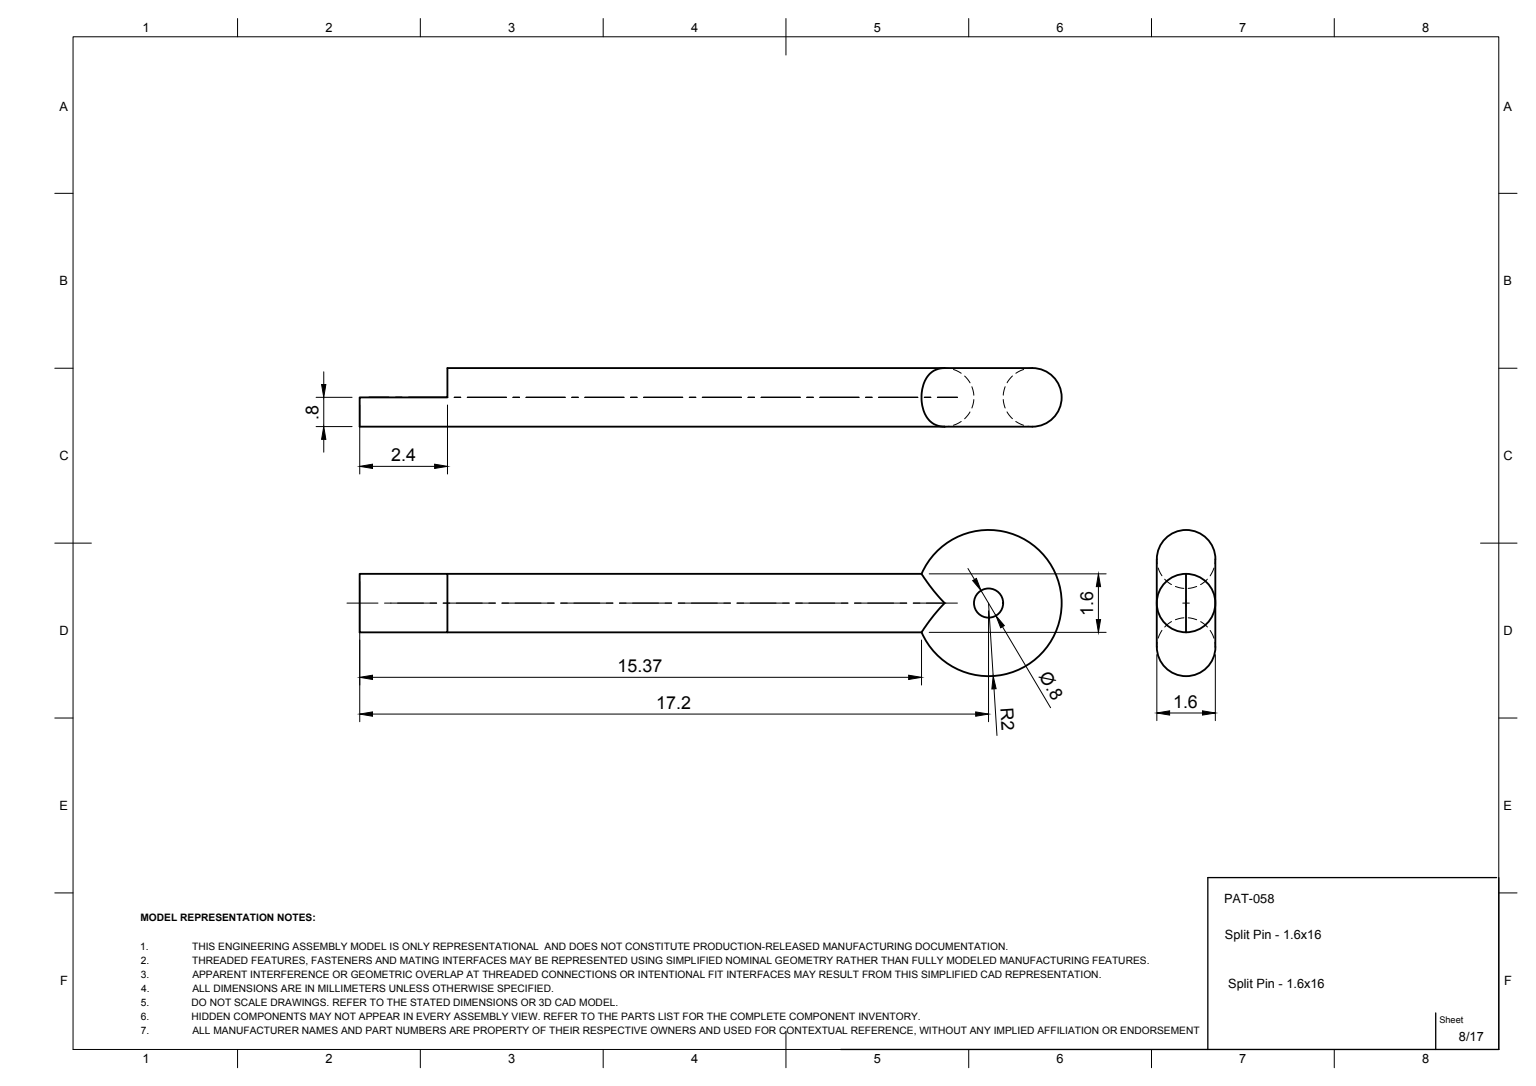
ISO-10303-21;
HEADER;
/* Generated by software containing ST-Developer
 * from STEP Tools, Inc. (www.steptools.com) 
 */

FILE_DESCRIPTION(
/* description */ ('Horizontal push-pull toggle clamp'),
/* implementation_level */ '2;1');

FILE_NAME(
/* name */ 'Split Pin - 1.6x16.step',
/* time_stamp */ '2026-10-27T21:21:09-07:00',
/* author */ (''),
/* organization */ (''),
/* preprocessor_version */ 'ST-DEVELOPER v20.2',
/* originating_system */ 'Autodesk Translation Framework v15.17.0.0',
/* authorisation */ '');

FILE_SCHEMA (('AUTOMOTIVE_DESIGN { 1 0 10303 214 3 1 1 }'));
ENDSEC;

DATA;
#10=MECHANICAL_DESIGN_GEOMETRIC_PRESENTATION_REPRESENTATION('',(#197),#4791);
#11=TOROIDAL_SURFACE('',#3033,0.12,0.08);
#16=B_SPLINE_CURVE_WITH_KNOTS('',3,(#4658,#4659,#4660,#4661,#4662,#4663,
#4664,#4665,#4666,#4667,#4668,#4669,#4670,#4671,#4672,#4673,#4674,#4675,
#4676,#4677,#4678,#4679,#4680,#4681,#4682,#4683),.UNSPECIFIED.,.F.,.F.,
(4,2,2,2,2,2,2,2,2,2,2,2,4),(-0.00054581412719389,0.,0.0281583564005144,
0.0618496465371181,0.0905865724114538,0.120694112793616,0.144966158459363,
0.16923820412511,0.199345744507272,0.228082670381608,0.261773960518212,
0.289932316918681,0.290478131045882),.UNSPECIFIED.);
#17=B_SPLINE_CURVE_WITH_KNOTS('',3,(#4684,#4685,#4686,#4687,#4688,#4689,
#4690,#4691,#4692,#4693,#4694,#4695,#4696,#4697,#4698,#4699,#4700,#4701,
#4702,#4703,#4704,#4705,#4706,#4707,#4708,#4709),.UNSPECIFIED.,.F.,.F.,
(4,2,2,2,2,2,2,2,2,2,2,2,4),(-0.000545814127196571,0.,0.0281583564006391,
0.0618496465374156,0.0905865724118984,0.120694112794215,0.144966158460086,
0.169238204125958,0.199345744508275,0.228082670382758,0.261773960519534,
0.289932316920171,0.29047813104737),.UNSPECIFIED.);
#171=SHAPE_REPRESENTATION_RELATIONSHIP('SRR','None',#4877,#184);
#184=ADVANCED_BREP_SHAPE_REPRESENTATION('',(#209),#4790);
#197=STYLED_ITEM('',(#5023),#209);
#209=MANIFOLD_SOLID_BREP('Body1',#2642);
#255=FACE_BOUND('',#705,.T.);
#359=PLANE('',#3036);
#360=PLANE('',#3038);
#361=PLANE('',#3042);
#508=FACE_OUTER_BOUND('',#704,.T.);
#509=FACE_OUTER_BOUND('',#706,.T.);
#510=FACE_OUTER_BOUND('',#707,.T.);
#511=FACE_OUTER_BOUND('',#708,.T.);
#512=FACE_OUTER_BOUND('',#709,.T.);
#704=EDGE_LOOP('',(#2419,#2420,#2421,#2422));
#705=EDGE_LOOP('',(#2423,#2424));
#706=EDGE_LOOP('',(#2425,#2426));
#707=EDGE_LOOP('',(#2427,#2428,#2429,#2430));
#708=EDGE_LOOP('',(#2431,#2432,#2433,#2434,#2435,#2436,#2437,#2438,#2439));
#709=EDGE_LOOP('',(#2440,#2441,#2442));
#791=CIRCLE('',#3034,0.08);
#792=CIRCLE('',#3035,0.04);
#793=CIRCLE('',#3037,0.08);
#794=CIRCLE('',#3040,0.08);
#795=CIRCLE('',#3041,0.08);
#1011=LINE('',#4714,#1231);
#1012=LINE('',#4717,#1232);
#1013=LINE('',#4719,#1233);
#1014=LINE('',#4720,#1234);
#1015=LINE('',#4724,#1235);
#1231=VECTOR('',#3787,1.);
#1232=VECTOR('',#3790,1.);
#1233=VECTOR('',#3791,1.);
#1234=VECTOR('',#3792,1.);
#1235=VECTOR('',#3797,0.08);
#1445=VERTEX_POINT('',#4653);
#1446=VERTEX_POINT('',#4656);
#1447=VERTEX_POINT('',#4657);
#1448=VERTEX_POINT('',#4711);
#1449=VERTEX_POINT('',#4712);
#1450=VERTEX_POINT('',#4716);
#1451=VERTEX_POINT('',#4718);
#1452=VERTEX_POINT('',#4722);
#1771=EDGE_CURVE('',#1445,#1445,#791,.T.);
#1772=EDGE_CURVE('',#1445,#1445,#792,.T.);
#1773=EDGE_CURVE('',#1446,#1447,#16,.T.);
#1774=EDGE_CURVE('',#1447,#1446,#17,.T.);
#1775=EDGE_CURVE('',#1448,#1449,#793,.T.);
#1776=EDGE_CURVE('',#1448,#1449,#1011,.T.);
#1777=EDGE_CURVE('',#1449,#1450,#1012,.T.);
#1778=EDGE_CURVE('',#1451,#1450,#1013,.T.);
#1779=EDGE_CURVE('',#1448,#1451,#1014,.T.);
#1780=EDGE_CURVE('',#1452,#1451,#794,.T.);
#1781=EDGE_CURVE('',#1452,#1447,#1015,.T.);
#1782=EDGE_CURVE('',#1450,#1452,#795,.T.);
#2419=ORIENTED_EDGE('',*,*,#1771,.F.);
#2420=ORIENTED_EDGE('',*,*,#1772,.T.);
#2421=ORIENTED_EDGE('',*,*,#1771,.T.);
#2422=ORIENTED_EDGE('',*,*,#1772,.F.);
#2423=ORIENTED_EDGE('',*,*,#1773,.F.);
#2424=ORIENTED_EDGE('',*,*,#1774,.F.);
#2425=ORIENTED_EDGE('',*,*,#1775,.T.);
#2426=ORIENTED_EDGE('',*,*,#1776,.F.);
#2427=ORIENTED_EDGE('',*,*,#1776,.T.);
#2428=ORIENTED_EDGE('',*,*,#1777,.T.);
#2429=ORIENTED_EDGE('',*,*,#1778,.F.);
#2430=ORIENTED_EDGE('',*,*,#1779,.F.);
#2431=ORIENTED_EDGE('',*,*,#1775,.F.);
#2432=ORIENTED_EDGE('',*,*,#1779,.T.);
#2433=ORIENTED_EDGE('',*,*,#1780,.F.);
#2434=ORIENTED_EDGE('',*,*,#1781,.T.);
#2435=ORIENTED_EDGE('',*,*,#1774,.T.);
#2436=ORIENTED_EDGE('',*,*,#1773,.T.);
#2437=ORIENTED_EDGE('',*,*,#1781,.F.);
#2438=ORIENTED_EDGE('',*,*,#1782,.F.);
#2439=ORIENTED_EDGE('',*,*,#1777,.F.);
#2440=ORIENTED_EDGE('',*,*,#1782,.T.);
#2441=ORIENTED_EDGE('',*,*,#1780,.T.);
#2442=ORIENTED_EDGE('',*,*,#1778,.T.);
#2477=CYLINDRICAL_SURFACE('',#3039,0.08);
#2624=ADVANCED_FACE('',(#508,#255),#11,.T.);
#2625=ADVANCED_FACE('',(#509),#359,.F.);
#2626=ADVANCED_FACE('',(#510),#360,.T.);
#2627=ADVANCED_FACE('',(#511),#2477,.T.);
#2628=ADVANCED_FACE('',(#512),#361,.F.);
#2642=CLOSED_SHELL('',(#2624,#2625,#2626,#2627,#2628));
#3032=AXIS2_PLACEMENT_3D('',#4651,#3775,#3776);
#3033=AXIS2_PLACEMENT_3D('',#4652,#3777,#3778);
#3034=AXIS2_PLACEMENT_3D('',#4654,#3779,#3780);
#3035=AXIS2_PLACEMENT_3D('',#4655,#3781,#3782);
#3036=AXIS2_PLACEMENT_3D('',#4710,#3783,#3784);
#3037=AXIS2_PLACEMENT_3D('',#4713,#3785,#3786);
#3038=AXIS2_PLACEMENT_3D('',#4715,#3788,#3789);
#3039=AXIS2_PLACEMENT_3D('',#4721,#3793,#3794);
#3040=AXIS2_PLACEMENT_3D('',#4723,#3795,#3796);
#3041=AXIS2_PLACEMENT_3D('',#4725,#3798,#3799);
#3042=AXIS2_PLACEMENT_3D('',#4726,#3800,#3801);
#3775=DIRECTION('axis',(0.,0.,1.));
#3776=DIRECTION('refdir',(1.,0.,0.));
#3777=DIRECTION('center_axis',(-1.,0.,0.));
#3778=DIRECTION('ref_axis',(0.,0.,1.));
#3779=DIRECTION('center_axis',(0.,-1.,1.38777878078145E-16));
#3780=DIRECTION('ref_axis',(0.,-1.38777878078145E-16,-1.));
#3781=DIRECTION('center_axis',(1.,0.,0.));
#3782=DIRECTION('ref_axis',(0.,0.,1.));
#3783=DIRECTION('center_axis',(0.,1.,0.));
#3784=DIRECTION('ref_axis',(1.,0.,0.));
#3785=DIRECTION('center_axis',(0.,-1.,0.));
#3786=DIRECTION('ref_axis',(1.,0.,0.));
#3787=DIRECTION('',(0.,0.,1.));
#3788=DIRECTION('center_axis',(1.,0.,0.));
#3789=DIRECTION('ref_axis',(0.,0.,1.));
#3790=DIRECTION('',(0.,-1.,0.));
#3791=DIRECTION('',(0.,0.,1.));
#3792=DIRECTION('',(0.,-1.,0.));
#3793=DIRECTION('center_axis',(0.,-1.,0.));
#3794=DIRECTION('ref_axis',(1.,0.,0.));
#3795=DIRECTION('center_axis',(0.,-1.,0.));
#3796=DIRECTION('ref_axis',(1.,0.,0.));
#3797=DIRECTION('',(0.,1.,0.));
#3798=DIRECTION('center_axis',(0.,-1.,0.));
#3799=DIRECTION('ref_axis',(1.,0.,0.));
#3800=DIRECTION('center_axis',(0.,1.,0.));
#3801=DIRECTION('ref_axis',(1.,0.,0.));
#4651=CARTESIAN_POINT('',(0.,0.,0.));
#4652=CARTESIAN_POINT('Origin',(0.,0.12,0.));
#4653=CARTESIAN_POINT('',(-9.79717439317883E-18,0.12,-0.04));
#4654=CARTESIAN_POINT('Origin',(0.,0.12,-0.12));
#4655=CARTESIAN_POINT('Origin',(9.79717439317883E-18,0.12,0.));
#4656=CARTESIAN_POINT('',(0.08,-4.89858719658941E-18,7.34788079488412E-18));
#4657=CARTESIAN_POINT('',(-0.08,-4.89858719658941E-18,7.34788079488412E-18));
#4658=CARTESIAN_POINT('Ctrl Pts',(0.08,-4.89858719658941E-18,7.34788079488412E-18));
#4659=CARTESIAN_POINT('Ctrl Pts',(0.08,-0.00012864962353541,0.000128649623535413));
#4660=CARTESIAN_POINT('Ctrl Pts',(0.0799996896739287,-0.00025719571182076,
0.000257402596003253));
#4661=CARTESIAN_POINT('Ctrl Pts',(0.0799669711262291,-0.00701193164572964,
0.00703384588894362));
#4662=CARTESIAN_POINT('Ctrl Pts',(0.0791054994909294,-0.0133457972655825,
0.0139383126556792));
#4663=CARTESIAN_POINT('Ctrl Pts',(0.0749700088488058,-0.0265076530862524,
0.0292212026164895));
#4664=CARTESIAN_POINT('Ctrl Pts',(0.0712702072865517,-0.0331317062461458,
0.0375603420117568));
#4665=CARTESIAN_POINT('Ctrl Pts',(0.0612858949407667,-0.0440683985740427,
0.0520545604187517));
#4666=CARTESIAN_POINT('Ctrl Pts',(0.0555090276731744,-0.0485199197794574,
0.0582717815295611));
#4667=CARTESIAN_POINT('Ctrl Pts',(0.0412398082144208,-0.0561090538733877,
0.0691638397919718));
#4668=CARTESIAN_POINT('Ctrl Pts',(0.0327878980890048,-0.059089642483296,
0.0736229049587921));
#4669=CARTESIAN_POINT('Ctrl Pts',(0.0159233027310102,-0.0625179833270725,
0.0787936360751706));
#4670=CARTESIAN_POINT('Ctrl Pts',(0.00801661414593076,-0.0633030277982336,
0.08));
#4671=CARTESIAN_POINT('Ctrl Pts',(-0.00801661414593074,-0.0633030277982336,
0.08));
#4672=CARTESIAN_POINT('Ctrl Pts',(-0.0159233027310102,-0.0625179833270726,
0.0787936360751706));
#4673=CARTESIAN_POINT('Ctrl Pts',(-0.0327878980890049,-0.059089642483296,
0.0736229049587921));
#4674=CARTESIAN_POINT('Ctrl Pts',(-0.0412398082144209,-0.0561090538733877,
0.0691638397919717));
#4675=CARTESIAN_POINT('Ctrl Pts',(-0.0555090276731744,-0.0485199197794574,
0.0582717815295611));
#4676=CARTESIAN_POINT('Ctrl Pts',(-0.0612858949407667,-0.0440683985740427,
0.0520545604187517));
#4677=CARTESIAN_POINT('Ctrl Pts',(-0.0712702072865517,-0.0331317062461458,
0.0375603420117568));
#4678=CARTESIAN_POINT('Ctrl Pts',(-0.0749700088488058,-0.0265076530862524,
0.0292212026164895));
#4679=CARTESIAN_POINT('Ctrl Pts',(-0.0791054994909264,-0.0133457972655921,
0.0139383126556903));
#4680=CARTESIAN_POINT('Ctrl Pts',(-0.0799669711262287,-0.00701193164579759,
0.0070338458890125));
#4681=CARTESIAN_POINT('Ctrl Pts',(-0.0799996896739287,-0.000257195711817665,
0.000257402596000083));
#4682=CARTESIAN_POINT('Ctrl Pts',(-0.08,-0.000128649623538514,0.000128649623538516));
#4683=CARTESIAN_POINT('Ctrl Pts',(-0.08,-4.89858719658941E-18,7.34788079488412E-18));
#4684=CARTESIAN_POINT('Ctrl Pts',(-0.08,-4.89858719658941E-18,7.34788079488412E-18));
#4685=CARTESIAN_POINT('Ctrl Pts',(-0.08,-0.000128649623536042,-0.00012864962353603));
#4686=CARTESIAN_POINT('Ctrl Pts',(-0.0799996896739287,-0.000257195711820127,
-0.000257402596002604));
#4687=CARTESIAN_POINT('Ctrl Pts',(-0.0799669711262289,-0.0070119316457589,
-0.00703384588897312));
#4688=CARTESIAN_POINT('Ctrl Pts',(-0.0791054994909281,-0.0133457972655867,
-0.0139383126556841));
#4689=CARTESIAN_POINT('Ctrl Pts',(-0.0749700088488058,-0.0265076530862525,
-0.0292212026164896));
#4690=CARTESIAN_POINT('Ctrl Pts',(-0.0712702072865516,-0.0331317062461459,
-0.0375603420117568));
#4691=CARTESIAN_POINT('Ctrl Pts',(-0.0612858949407667,-0.0440683985740427,
-0.0520545604187517));
#4692=CARTESIAN_POINT('Ctrl Pts',(-0.0555090276731744,-0.0485199197794574,
-0.0582717815295611));
#4693=CARTESIAN_POINT('Ctrl Pts',(-0.0412398082144209,-0.0561090538733877,
-0.0691638397919717));
#4694=CARTESIAN_POINT('Ctrl Pts',(-0.0327878980890049,-0.059089642483296,
-0.0736229049587921));
#4695=CARTESIAN_POINT('Ctrl Pts',(-0.0159233027310101,-0.0625179833270725,
-0.0787936360751706));
#4696=CARTESIAN_POINT('Ctrl Pts',(-0.00801661414593069,-0.0633030277982336,
-0.08));
#4697=CARTESIAN_POINT('Ctrl Pts',(0.0080166141459307,-0.0633030277982336,
-0.08));
#4698=CARTESIAN_POINT('Ctrl Pts',(0.0159233027310101,-0.0625179833270725,
-0.0787936360751706));
#4699=CARTESIAN_POINT('Ctrl Pts',(0.0327878980890049,-0.0590896424832959,
-0.0736229049587921));
#4700=CARTESIAN_POINT('Ctrl Pts',(0.0412398082144209,-0.0561090538733877,
-0.0691638397919717));
#4701=CARTESIAN_POINT('Ctrl Pts',(0.0555090276731744,-0.0485199197794574,
-0.0582717815295611));
#4702=CARTESIAN_POINT('Ctrl Pts',(0.0612858949407666,-0.0440683985740428,
-0.0520545604187518));
#4703=CARTESIAN_POINT('Ctrl Pts',(0.0712702072865517,-0.0331317062461458,
-0.0375603420117568));
#4704=CARTESIAN_POINT('Ctrl Pts',(0.0749700088488058,-0.0265076530862524,
-0.0292212026164895));
#4705=CARTESIAN_POINT('Ctrl Pts',(0.079105499490928,-0.013345797265587,
-0.0139383126556845));
#4706=CARTESIAN_POINT('Ctrl Pts',(0.0799669711262289,-0.00701193164576148,
-0.00703384588897579));
#4707=CARTESIAN_POINT('Ctrl Pts',(0.0799996896739287,-0.000257195711819584,
-0.000257402596002039));
#4708=CARTESIAN_POINT('Ctrl Pts',(0.08,-0.000128649623536605,-0.000128649623536593));
#4709=CARTESIAN_POINT('Ctrl Pts',(0.08,-4.89858719658941E-18,7.34788079488412E-18));
#4710=CARTESIAN_POINT('Origin',(0.04,-1.36,0.));
#4711=CARTESIAN_POINT('',(0.,-1.36,-0.08));
#4712=CARTESIAN_POINT('',(0.,-1.36,0.08));
#4713=CARTESIAN_POINT('Origin',(0.,-1.36,0.));
#4714=CARTESIAN_POINT('',(0.,-1.36,-0.04));
#4715=CARTESIAN_POINT('Origin',(0.,0.,-0.08));
#4716=CARTESIAN_POINT('',(0.,-1.6,0.08));
#4717=CARTESIAN_POINT('',(0.,0.,0.08));
#4718=CARTESIAN_POINT('',(0.,-1.6,-0.08));
#4719=CARTESIAN_POINT('',(0.,-1.6,-0.09));
#4720=CARTESIAN_POINT('',(0.,0.,-0.08));
#4721=CARTESIAN_POINT('Origin',(0.,0.,0.));
#4722=CARTESIAN_POINT('',(-0.08,-1.6,-9.79717439317883E-18));
#4723=CARTESIAN_POINT('Origin',(0.,-1.6,0.));
#4724=CARTESIAN_POINT('',(-0.08,0.,-9.79717439317883E-18));
#4725=CARTESIAN_POINT('Origin',(0.,-1.6,0.));
#4726=CARTESIAN_POINT('Origin',(-0.04,-1.6,0.));
#4771=UNCERTAINTY_MEASURE_WITH_UNIT(LENGTH_MEASURE(0.001),#4792,
'DISTANCE_ACCURACY_VALUE',
'Maximum model space distance between geometric entities at asserted c
onnectivities');
#4772=UNCERTAINTY_MEASURE_WITH_UNIT(LENGTH_MEASURE(0.001),#4792,
'DISTANCE_ACCURACY_VALUE',
'Maximum model space distance between geometric entities at asserted c
onnectivities');
#4790=(
GEOMETRIC_REPRESENTATION_CONTEXT(3)
GLOBAL_UNCERTAINTY_ASSIGNED_CONTEXT((#4771))
GLOBAL_UNIT_ASSIGNED_CONTEXT((#4792,#4794,#4795))
REPRESENTATION_CONTEXT('','3D')
);
#4791=(
GEOMETRIC_REPRESENTATION_CONTEXT(3)
GLOBAL_UNCERTAINTY_ASSIGNED_CONTEXT((#4772))
GLOBAL_UNIT_ASSIGNED_CONTEXT((#4792,#4794,#4795))
REPRESENTATION_CONTEXT('','3D')
);
#4792=(
LENGTH_UNIT()
NAMED_UNIT(*)
SI_UNIT(.CENTI.,.METRE.)
);
#4794=(
NAMED_UNIT(*)
PLANE_ANGLE_UNIT()
SI_UNIT($,.RADIAN.)
);
#4795=(
NAMED_UNIT(*)
SI_UNIT($,.STERADIAN.)
SOLID_ANGLE_UNIT()
);
#4813=SHAPE_DEFINITION_REPRESENTATION(#4832,#4877);
#4832=PRODUCT_DEFINITION_SHAPE('',$,#4896);
#4877=SHAPE_REPRESENTATION('',(#3032),#4790);
#4878=PRODUCT_DEFINITION_CONTEXT('part definition',#4934,'design');
#4896=PRODUCT_DEFINITION('Split Pin - 1.6x16','Split Pin - 1.6x16',#4914,
#4878);
#4914=PRODUCT_DEFINITION_FORMATION('',$,#4953);
#4934=APPLICATION_CONTEXT(
'Core Data for Automotive Mechanical Design Process');
#4935=PRODUCT_CONTEXT('part definition',#4934,'mechanical');
#4953=PRODUCT('Split Pin - 1.6x16','Split Pin - 1.6x16',
'Split Pin - 1.6x16',(#4935));
#5017=COLOUR_RGB('Grey',0.48,0.52,0.57);
#5018=FILL_AREA_STYLE_COLOUR('',#5017);
#5019=FILL_AREA_STYLE('',(#5018));
#5020=SURFACE_STYLE_FILL_AREA(#5019);
#5021=SURFACE_SIDE_STYLE('',(#5020));
#5022=SURFACE_STYLE_USAGE(.BOTH.,#5021);
#5023=PRESENTATION_STYLE_ASSIGNMENT((#5022));
ENDSEC;
END-ISO-10303-21;
